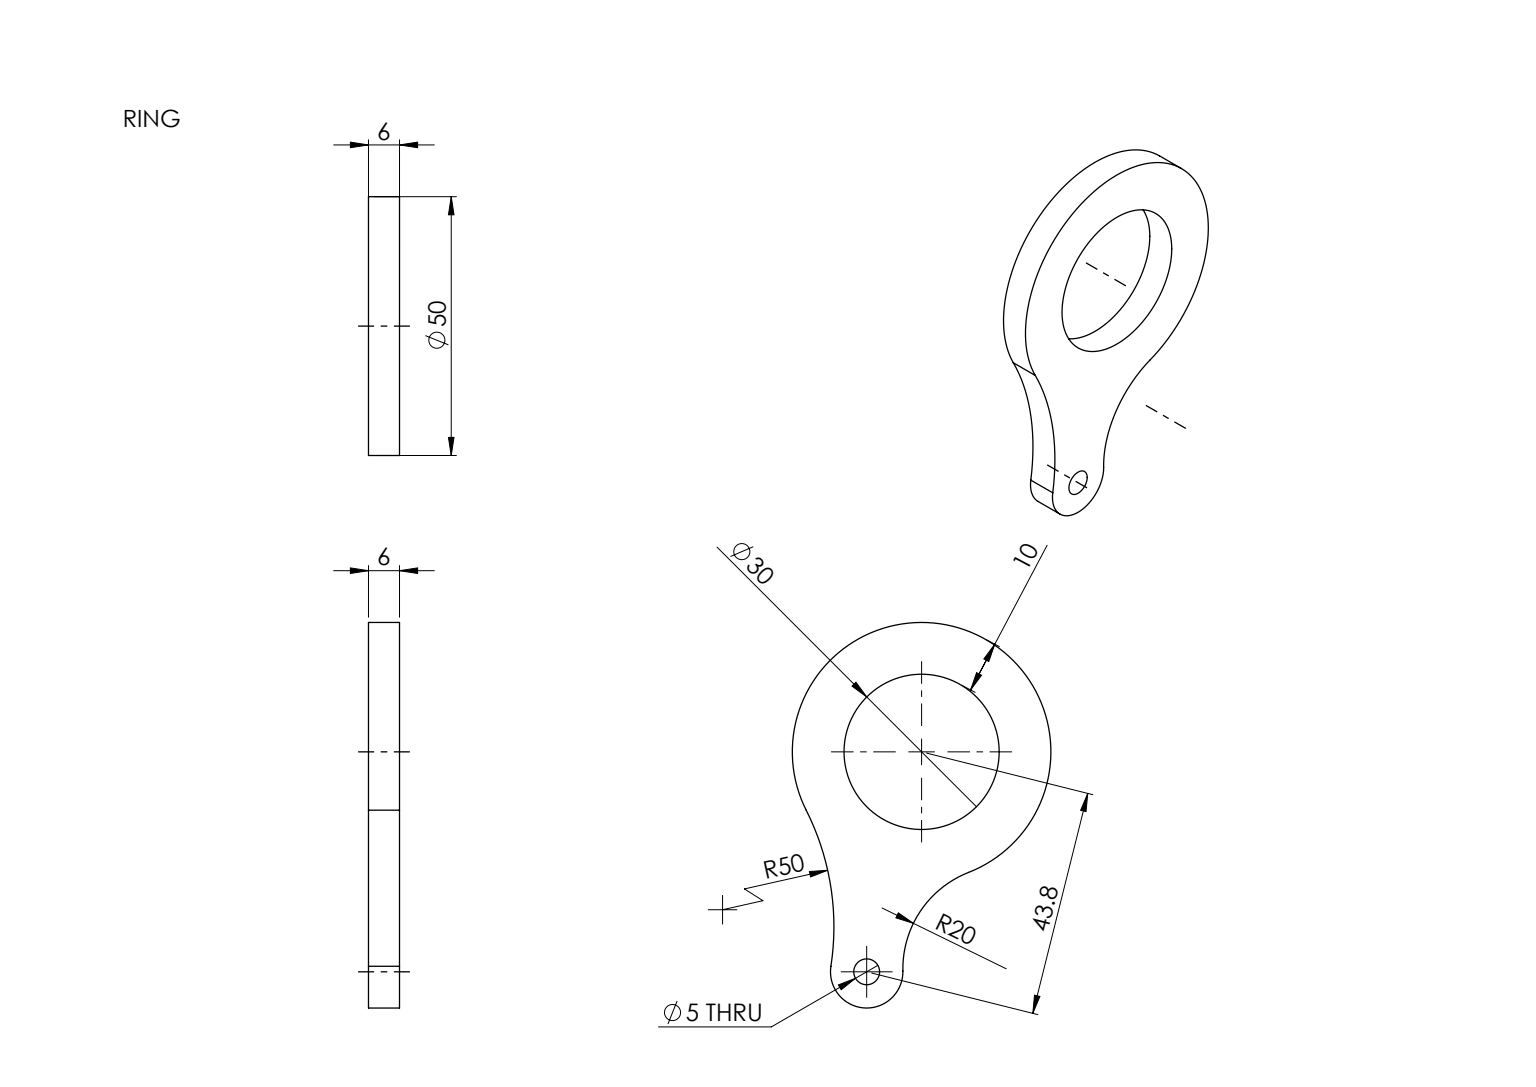
ISO-10303-21;
HEADER;
FILE_DESCRIPTION (('STEP AP214'),
    '1' );
FILE_NAME ('ring.step',
    '2026-10-03T20:08:58',
    ( '' ),
    ( '' ),
    'SwSTEP 2.0',
    'SolidWorks 2026',
    '' );
FILE_SCHEMA (( 'AUTOMOTIVE_DESIGN' ));
ENDSEC;

DATA;
#6=CARTESIAN_POINT ( 'NONE',  ( 33.00000000000001421, 39.34792583643766761, -10.06347054209568270 ) ) ;
#20=( GEOMETRIC_REPRESENTATION_CONTEXT ( 3 ) GLOBAL_UNCERTAINTY_ASSIGNED_CONTEXT ( ( #3670 ) ) GLOBAL_UNIT_ASSIGNED_CONTEXT ( ( #5671, #4709, #1872 ) ) REPRESENTATION_CONTEXT ( 'NONE', 'WORKASPACE' ) );
#46=EDGE_CURVE ( 'NONE', #9407, #3079, #7991, .T. ) ;
#83=ORIENTED_EDGE ( 'NONE', *, *, #1095, .T. ) ;
#164=EDGE_CURVE ( 'NONE', #2848, #3887, #6852, .T. ) ;
#223=EDGE_LOOP ( 'NONE', ( #680, #8634, #6232, #8801 ) ) ;
#258=AXIS2_PLACEMENT_3D ( 'NONE', #11847, #1979, #9819 ) ;
#260=CARTESIAN_POINT ( 'NONE',  ( 33.00000000000001421, 39.34792583643766761, -17.06347054209568270 ) ) ;
#266=DIRECTION ( 'NONE',  ( -1.000000000000000000, 1.006188713385347367E-17, 3.844790828812615713E-17 ) ) ;
#269=EDGE_CURVE ( 'NONE', #1961, #1191, #3966, .T. ) ;
#278=AXIS2_PLACEMENT_3D ( 'NONE', #6450, #2458, #6380 ) ;
#348=ORIENTED_EDGE ( 'NONE', *, *, #8128, .T. ) ;
#366=DIRECTION ( 'NONE',  ( -1.000000000000000000, 1.006188713385347367E-17, 3.844790828812615713E-17 ) ) ;
#371=CARTESIAN_POINT ( 'NONE',  ( 33.00000000000001421, 81.84122341717352356, -52.68198508464163154 ) ) ;
#423=CARTESIAN_POINT ( 'NONE',  ( 33.00000000000000711, 58.55522666905708462, -36.77936687539386185 ) ) ;
#426=DIRECTION ( 'NONE',  ( 1.000000000000000000, -6.162975822039154730E-33, -4.563833282352349791E-17 ) ) ;
#428=ORIENTED_EDGE ( 'NONE', *, *, #736, .F. ) ;
#451=CARTESIAN_POINT ( 'NONE',  ( 33.00000000000001421, 81.84122341717352356, -27.68198508464163510 ) ) ;
#457=ORIENTED_EDGE ( 'NONE', *, *, #9263, .T. ) ;
#554=DIRECTION ( 'NONE',  ( 1.000000000000000000, -6.162975822039154730E-33, -4.563833282352349791E-17 ) ) ;
#581=CARTESIAN_POINT ( 'NONE',  ( 27.00000000000001421, 39.34792583643766761, -17.06347054209568270 ) ) ;
#597=CIRCLE ( 'NONE', #1831, 24.99999999999998934 ) ;
#631=LINE ( 'NONE', #12621, #6264 ) ;
#666=EDGE_CURVE ( 'NONE', #10338, #2092, #3944, .T. ) ;
#676=PLANE ( 'NONE',  #3004 ) ;
#680=ORIENTED_EDGE ( 'NONE', *, *, #6194, .F. ) ;
#735=CYLINDRICAL_SURFACE ( 'NONE', #7583, 19.99999999999999645 ) ;
#736=EDGE_CURVE ( 'NONE', #1153, #9287, #7907, .T. ) ;
#748=EDGE_LOOP ( 'NONE', ( #2877, #7113, #11794, #1502 ) ) ;
#794=CARTESIAN_POINT ( 'NONE',  ( 33.00000000000001421, 40.41548023366553366, -10.14535464186970870 ) ) ;
#795=FACE_BOUND ( 'NONE', #2630, .T. ) ;
#840=EDGE_CURVE ( 'NONE', #1206, #1961, #10652, .T. ) ;
#886=ORIENTED_EDGE ( 'NONE', *, *, #164, .F. ) ;
#890=FACE_OUTER_BOUND ( 'NONE', #6082, .T. ) ;
#900=ORIENTED_EDGE ( 'NONE', *, *, #1095, .F. ) ;
#947=ORIENTED_EDGE ( 'NONE', *, *, #1314, .T. ) ;
#1023=CARTESIAN_POINT ( 'NONE',  ( 33.00000000000000711, 39.92642927056392210, -24.05727230799563898 ) ) ;
#1028=AXIS2_PLACEMENT_3D ( 'NONE', #11252, #426, #7264 ) ;
#1036=LINE ( 'NONE', #4975, #8822 ) ;
#1043=DIRECTION ( 'NONE',  ( 1.000000000000000000, -6.162975822039154730E-33, -4.563833282352349791E-17 ) ) ;
#1082=CIRCLE ( 'NONE', #2757, 19.99999999999998934 ) ;
#1095=EDGE_CURVE ( 'NONE', #3948, #3079, #5308, .T. ) ;
#1107=FACE_OUTER_BOUND ( 'NONE', #1947, .T. ) ;
#1129=ADVANCED_FACE ( 'NONE', ( #11502 ), #735, .F. ) ;
#1153=VERTEX_POINT ( 'NONE', #9602 ) ;
#1170=DIRECTION ( 'NONE',  ( 0.000000000000000000, 0.000000000000000000, -1.000000000000000000 ) ) ;
#1191=VERTEX_POINT ( 'NONE', #794 ) ;
#1206=VERTEX_POINT ( 'NONE', #2693 ) ;
#1215=EDGE_LOOP ( 'NONE', ( #8140, #5838, #6921, #7199 ) ) ;
#1239=CYLINDRICAL_SURFACE ( 'NONE', #2419, 14.99999999999998757 ) ;
#1257=CARTESIAN_POINT ( 'NONE',  ( 27.00000000000001421, 39.49790820824818383, -24.06186359251418594 ) ) ;
#1314=EDGE_CURVE ( 'NONE', #2160, #10794, #1409, .T. ) ;
#1319=DIRECTION ( 'NONE',  ( 0.000000000000000000, 0.000000000000000000, 1.000000000000000000 ) ) ;
#1336=AXIS2_PLACEMENT_3D ( 'NONE', #3651, #3590, #11505 ) ;
#1362=DIRECTION ( 'NONE',  ( 0.000000000000000000, 0.000000000000000000, -1.000000000000000000 ) ) ;
#1372=ORIENTED_EDGE ( 'NONE', *, *, #11676, .T. ) ;
#1383=CARTESIAN_POINT ( 'NONE',  ( 33.00000000000001421, 48.04086878529346194, 39.26975893117280947 ) ) ;
#1409=CIRCLE ( 'NONE', #3880, 2.499999999999992006 ) ;
#1440=ORIENTED_EDGE ( 'NONE', *, *, #12668, .F. ) ;
#1449=CYLINDRICAL_SURFACE ( 'NONE', #6515, 49.99999999999995026 ) ;
#1487=VECTOR ( 'NONE', #10109, 1000.000000000000000 ) ;
#1502=ORIENTED_EDGE ( 'NONE', *, *, #10839, .F. ) ;
#1510=FILL_AREA_STYLE ('',( #7502 ) ) ;
#1512=DIRECTION ( 'NONE',  ( 0.000000000000000000, 0.000000000000000000, 1.000000000000000000 ) ) ;
#1520=DIRECTION ( 'NONE',  ( 0.000000000000000000, 0.000000000000000000, -1.000000000000000000 ) ) ;
#1532=CIRCLE ( 'NONE', #9136, 14.99999999999998934 ) ;
#1539=VECTOR ( 'NONE', #5857, 1000.000000000000000 ) ;
#1606=DIRECTION ( 'NONE',  ( 1.000000000000000000, -6.162975822039154730E-33, -4.563833282352349791E-17 ) ) ;
#1617=AXIS2_PLACEMENT_3D ( 'NONE', #11073, #11142, #1520 ) ;
#1624=DIRECTION ( 'NONE',  ( 0.000000000000000000, 0.000000000000000000, 1.000000000000000000 ) ) ;
#1634=ORIENTED_EDGE ( 'NONE', *, *, #6345, .F. ) ;
#1653=CIRCLE ( 'NONE', #1617, 6.999999999999999112 ) ;
#1671=MECHANICAL_DESIGN_GEOMETRIC_PRESENTATION_REPRESENTATION('',(#4964),#9261);
#1679=DIRECTION ( 'NONE',  ( 1.000000000000000000, -6.162975822039154730E-33, -4.563833282352349791E-17 ) ) ;
#1707=CARTESIAN_POINT ( 'NONE',  ( 27.00000000000001421, 81.84122341717352356, -27.68198508464163510 ) ) ;
#1728=UNCERTAINTY_MEASURE_WITH_UNIT (LENGTH_MEASURE( 1.000000000000000082E-05 ), #6656, 'distance_accuracy_value', 'NONE');
#1732=APPLICATION_CONTEXT ( 'automotive_design' ) ;
#1739=ADVANCED_BREP_SHAPE_REPRESENTATION ( '', ( #5956, #12422 ), #20 ) ;
#1753=DIRECTION ( 'NONE',  ( 0.000000000000000000, 0.000000000000000000, 1.000000000000000000 ) ) ;
#1754=CIRCLE ( 'NONE', #4433, 24.99999999999998934 ) ;
#1825=( LENGTH_UNIT ( ) NAMED_UNIT ( * ) SI_UNIT ( .MILLI., .METRE. ) );
#1831=AXIS2_PLACEMENT_3D ( 'NONE', #8871, #4958, #6761 ) ;
#1872=( NAMED_UNIT ( * ) SI_UNIT ( $, .STERADIAN. ) SOLID_ANGLE_UNIT ( ) );
#1891=DIRECTION ( 'NONE',  ( -4.563833282352349791E-17, 0.000000000000000000, -1.000000000000000000 ) ) ;
#1921=CARTESIAN_POINT ( 'NONE',  ( 33.00000000000001421, 39.34792583643766761, -17.06347054209568270 ) ) ;
#1947=EDGE_LOOP ( 'NONE', ( #8020, #6144, #3063, #8330 ) ) ;
#1957=CARTESIAN_POINT ( 'NONE',  ( 27.00000000000001421, 81.84122341717352356, -27.68198508464163510 ) ) ;
#1959=ORIENTED_EDGE ( 'NONE', *, *, #8551, .T. ) ;
#1961=VERTEX_POINT ( 'NONE', #4156 ) ;
#1979=DIRECTION ( 'NONE',  ( -1.000000000000000000, 6.162975822039154730E-33, 4.563833282352349791E-17 ) ) ;
#2050=EDGE_LOOP ( 'NONE', ( #8866, #9247, #9932, #4731 ) ) ;
#2056=LINE ( 'NONE', #5982, #6902 ) ;
#2089=DIRECTION ( 'NONE',  ( 0.000000000000000000, 0.000000000000000000, -1.000000000000000000 ) ) ;
#2092=VERTEX_POINT ( 'NONE', #9392 ) ;
#2128=CARTESIAN_POINT ( 'NONE',  ( 33.00000000000001421, 39.34792583643766761, -19.56347054209567204 ) ) ;
#2150=DIRECTION ( 'NONE',  ( -1.000000000000000000, 1.006188713385347367E-17, 3.844790828812615713E-17 ) ) ;
#2160=VERTEX_POINT ( 'NONE', #5421 ) ;
#2198=CARTESIAN_POINT ( 'NONE',  ( 33.00000000000001421, 81.84122341717352356, -27.68198508464163510 ) ) ;
#2210=PRODUCT_DEFINITION_FORMATION_WITH_SPECIFIED_SOURCE ( 'ANY', '', #4538, .NOT_KNOWN. ) ;
#2241=EDGE_CURVE ( 'NONE', #4528, #5879, #11115, .T. ) ;
#2250=ORIENTED_EDGE ( 'NONE', *, *, #666, .F. ) ;
#2346=CARTESIAN_POINT ( 'NONE',  ( 27.00000000000001421, 81.84122341717352356, -27.68198508464163510 ) ) ;
#2360=CARTESIAN_POINT ( 'NONE',  ( 33.00000000000001421, 70.57443853988016258, -5.364737079370081041 ) ) ;
#2380=LINE ( 'NONE', #4172, #2959 ) ;
#2412=DIRECTION ( 'NONE',  ( 0.000000000000000000, 0.000000000000000000, 1.000000000000000000 ) ) ;
#2419=AXIS2_PLACEMENT_3D ( 'NONE', #11230, #2150, #2412 ) ;
#2446=LINE ( 'NONE', #11331, #4270 ) ;
#2458=DIRECTION ( 'NONE',  ( -1.000000000000000000, 6.162975822039154730E-33, 4.563833282352349791E-17 ) ) ;
#2539=ORIENTED_EDGE ( 'NONE', *, *, #10803, .F. ) ;
#2548=DIRECTION ( 'NONE',  ( -1.000000000000000000, 1.006188713385347367E-17, 3.844790828812615713E-17 ) ) ;
#2555=DIRECTION ( 'NONE',  ( 0.000000000000000000, 0.000000000000000000, 1.000000000000000000 ) ) ;
#2558=CARTESIAN_POINT ( 'NONE',  ( 33.00000000000001421, -6.037132280312101458E-17, -1.462922435963892052E-15 ) ) ;
#2609=UNCERTAINTY_MEASURE_WITH_UNIT (LENGTH_MEASURE( 1.000000000000000082E-05 ), #1825, 'distance_accuracy_value', 'NONE');
#2630=EDGE_LOOP ( 'NONE', ( #457, #9132 ) ) ;
#2669=EDGE_CURVE ( 'NONE', #7265, #2754, #597, .T. ) ;
#2678=ADVANCED_FACE ( 'NONE', ( #890 ), #10614, .F. ) ;
#2693=CARTESIAN_POINT ( 'NONE',  ( 33.00000000000001421, 81.84122341717352356, -2.681985084641642203 ) ) ;
#2711=EDGE_LOOP ( 'NONE', ( #11837, #7268, #900, #4477 ) ) ;
#2720=ORIENTED_EDGE ( 'NONE', *, *, #840, .F. ) ;
#2726=SHAPE_REPRESENTATION ( 'ring', ( #12422 ), #20 ) ;
#2734=VERTEX_POINT ( 'NONE', #7273 ) ;
#2736=( NAMED_UNIT ( * ) SI_UNIT ( $, .STERADIAN. ) SOLID_ANGLE_UNIT ( ) );
#2738=AXIS2_PLACEMENT_3D ( 'NONE', #4200, #4008, #1170 ) ;
#2754=VERTEX_POINT ( 'NONE', #371 ) ;
#2757=AXIS2_PLACEMENT_3D ( 'NONE', #11977, #10733, #4955 ) ;
#2761=CARTESIAN_POINT ( 'NONE',  ( 27.00000000000001421, -1.664003471950572653E-31, -1.232234986235134900E-15 ) ) ;
#2788=ORIENTED_EDGE ( 'NONE', *, *, #12668, .T. ) ;
#2795=ORIENTED_EDGE ( 'NONE', *, *, #2241, .F. ) ;
#2806=CARTESIAN_POINT ( 'NONE',  ( 33.00000000000001421, 39.34792583643766761, -17.06347054209568270 ) ) ;
#2848=VERTEX_POINT ( 'NONE', #11392 ) ;
#2867=CARTESIAN_POINT ( 'NONE',  ( 27.00000000000001066, 39.92642927056392210, -44.05727230799563898 ) ) ;
#2877=ORIENTED_EDGE ( 'NONE', *, *, #9073, .F. ) ;
#2929=DIRECTION ( 'NONE',  ( -1.000000000000000000, 1.006188713385347367E-17, 3.844790828812615713E-17 ) ) ;
#2959=VECTOR ( 'NONE', #366, 1000.000000000000000 ) ;
#2981=AXIS2_PLACEMENT_3D ( 'NONE', #2867, #7614, #11554 ) ;
#2984=DIRECTION ( 'NONE',  ( 0.000000000000000000, 0.000000000000000000, -1.000000000000000000 ) ) ;
#3004=AXIS2_PLACEMENT_3D ( 'NONE', #2558, #554, #5699 ) ;
#3027=ORIENTED_EDGE ( 'NONE', *, *, #2241, .T. ) ;
#3040=EDGE_CURVE ( 'NONE', #5879, #8571, #4201, .T. ) ;
#3050=CYLINDRICAL_SURFACE ( 'NONE', #12197, 24.99999999999999289 ) ;
#3061=APPLICATION_CONTEXT ( 'automotive_design' ) ;
#3063=ORIENTED_EDGE ( 'NONE', *, *, #6754, .T. ) ;
#3079=VERTEX_POINT ( 'NONE', #8800 ) ;
#3127=CARTESIAN_POINT ( 'NONE',  ( 33.00000000000000711, 39.92642927056392210, -24.05727230799563898 ) ) ;
#3185=DIRECTION ( 'NONE',  ( 0.000000000000000000, 0.000000000000000000, 1.000000000000000000 ) ) ;
#3211=EDGE_LOOP ( 'NONE', ( #2720, #3521, #1959, #7626 ) ) ;
#3269=ORIENTED_EDGE ( 'NONE', *, *, #10839, .T. ) ;
#3353=ORIENTED_EDGE ( 'NONE', *, *, #12439, .F. ) ;
#3398=ORIENTED_EDGE ( 'NONE', *, *, #10467, .F. ) ;
#3451=AXIS2_PLACEMENT_3D ( 'NONE', #2806, #10632, #1753 ) ;
#3456=DIRECTION ( 'NONE',  ( -1.000000000000000000, 1.006188713385347367E-17, 3.844790828812615713E-17 ) ) ;
#3462=AXIS2_PLACEMENT_3D ( 'NONE', #7581, #11525, #6631 ) ;
#3517=CYLINDRICAL_SURFACE ( 'NONE', #8257, 24.99999999999999289 ) ;
#3521=ORIENTED_EDGE ( 'NONE', *, *, #8172, .T. ) ;
#3583=ADVANCED_FACE ( 'NONE', ( #1107 ), #5235, .F. ) ;
#3590=DIRECTION ( 'NONE',  ( -1.000000000000000000, 1.006188713385347367E-17, 3.844790828812615713E-17 ) ) ;
#3631=DIRECTION ( 'NONE',  ( 0.000000000000000000, 0.000000000000000000, -1.000000000000000000 ) ) ;
#3651=CARTESIAN_POINT ( 'NONE',  ( 33.00000000000001421, 39.34792583643766761, -17.06347054209568270 ) ) ;
#3670=UNCERTAINTY_MEASURE_WITH_UNIT (LENGTH_MEASURE( 1.000000000000000082E-05 ), #5671, 'distance_accuracy_value', 'NONE');
#3756=DIRECTION ( 'NONE',  ( 1.000000000000000000, -6.162975822039154730E-33, -4.563833282352349791E-17 ) ) ;
#3769=DIRECTION ( 'NONE',  ( 1.000000000000000000, -6.162975822039154730E-33, -4.563833282352349791E-17 ) ) ;
#3780=VERTEX_POINT ( 'NONE', #9278 ) ;
#3781=ORIENTED_EDGE ( 'NONE', *, *, #8551, .F. ) ;
#3834=AXIS2_PLACEMENT_3D ( 'NONE', #7565, #10323, #1512 ) ;
#3851=DIRECTION ( 'NONE',  ( 0.000000000000000000, 0.000000000000000000, -1.000000000000000000 ) ) ;
#3880=AXIS2_PLACEMENT_3D ( 'NONE', #9858, #1043, #8964 ) ;
#3887=VERTEX_POINT ( 'NONE', #12646 ) ;
#3889=( NAMED_UNIT ( * ) SI_UNIT ( $, .STERADIAN. ) SOLID_ANGLE_UNIT ( ) );
#3917=CIRCLE ( 'NONE', #4535, 24.99999999999998934 ) ;
#3944=CIRCLE ( 'NONE', #7444, 14.99999999999998934 ) ;
#3948=VERTEX_POINT ( 'NONE', #4655 ) ;
#3966=CIRCLE ( 'NONE', #11164, 49.99999999999994316 ) ;
#3969=EDGE_CURVE ( 'NONE', #3079, #4528, #6047, .T. ) ;
#4008=DIRECTION ( 'NONE',  ( -1.000000000000000000, 6.162975822039154730E-33, 4.563833282352349791E-17 ) ) ;
#4047=VECTOR ( 'NONE', #6397, 1000.000000000000000 ) ;
#4156=CARTESIAN_POINT ( 'NONE',  ( 33.00000000000001421, 70.57443853988016258, -5.364737079370081041 ) ) ;
#4172=CARTESIAN_POINT ( 'NONE',  ( 33.00000000000001421, 39.34792583643766761, -19.56347054209567204 ) ) ;
#4200=CARTESIAN_POINT ( 'NONE',  ( 33.00000000000001421, 39.34792583643766761, -17.06347054209568270 ) ) ;
#4201=CIRCLE ( 'NONE', #12027, 6.999999999999999112 ) ;
#4261=AXIS2_PLACEMENT_3D ( 'NONE', #260, #7098, #3185 ) ;
#4263=DIRECTION ( 'NONE',  ( -1.000000000000000000, 1.006188713385347367E-17, 3.844790828812615713E-17 ) ) ;
#4266=ADVANCED_FACE ( 'NONE', ( #4627 ), #8547, .F. ) ;
#4270=VECTOR ( 'NONE', #6881, 1000.000000000000000 ) ;
#4275=LINE ( 'NONE', #2360, #9888 ) ;
#4283=EDGE_CURVE ( 'NONE', #9287, #5879, #2446, .T. ) ;
#4315=VECTOR ( 'NONE', #266, 1000.000000000000000 ) ;
#4341=ORIENTED_EDGE ( 'NONE', *, *, #164, .T. ) ;
#4381=CIRCLE ( 'NONE', #258, 6.999999999999999112 ) ;
#4405=ORIENTED_EDGE ( 'NONE', *, *, #840, .T. ) ;
#4433=AXIS2_PLACEMENT_3D ( 'NONE', #1707, #6549, #7636 ) ;
#4458=MECHANICAL_DESIGN_GEOMETRIC_PRESENTATION_REPRESENTATION('',(#7344),#10617);
#4477=ORIENTED_EDGE ( 'NONE', *, *, #4523, .F. ) ;
#4481=PRESENTATION_STYLE_ASSIGNMENT (( #9352 ) ) ;
#4493=VERTEX_POINT ( 'NONE', #8150 ) ;
#4523=EDGE_CURVE ( 'NONE', #7265, #3948, #11899, .T. ) ;
#4528=VERTEX_POINT ( 'NONE', #1257 ) ;
#4535=AXIS2_PLACEMENT_3D ( 'NONE', #9705, #7026, #2984 ) ;
#4538=PRODUCT ( 'ring', 'ring', '', ( #10781 ) ) ;
#4548=SURFACE_STYLE_FILL_AREA ( #1510 ) ;
#4619=EDGE_LOOP ( 'NONE', ( #4341, #12276 ) ) ;
#4627=FACE_OUTER_BOUND ( 'NONE', #2711, .T. ) ;
#4655=CARTESIAN_POINT ( 'NONE',  ( 27.00000000000001066, 58.55522666905708462, -36.77936687539386185 ) ) ;
#4660=ADVANCED_FACE ( 'NONE', ( #7445 ), #6613, .F. ) ;
#4671=AXIS2_PLACEMENT_3D ( 'NONE', #8322, #10306, #1624 ) ;
#4672=FACE_BOUND ( 'NONE', #4619, .T. ) ;
#4709=( NAMED_UNIT ( * ) PLANE_ANGLE_UNIT ( ) SI_UNIT ( $, .RADIAN. ) );
#4729=AXIS2_PLACEMENT_3D ( 'NONE', #11567, #3769, #8401 ) ;
#4731=ORIENTED_EDGE ( 'NONE', *, *, #8172, .F. ) ;
#4777=DIRECTION ( 'NONE',  ( 0.000000000000000000, 6.839766848137126197E-14, -1.000000000000000000 ) ) ;
#4824=ADVANCED_FACE ( 'NONE', ( #4672, #8724, #795 ), #7876, .F. ) ;
#4955=DIRECTION ( 'NONE',  ( 0.000000000000000000, 0.000000000000000000, -1.000000000000000000 ) ) ;
#4958=DIRECTION ( 'NONE',  ( 1.000000000000000000, -6.162975822039154730E-33, -4.563833282352349791E-17 ) ) ;
#4964=STYLED_ITEM ( 'NONE', ( #10686 ), #1739 ) ;
#4975=CARTESIAN_POINT ( 'NONE',  ( 33.00000000000001421, 39.34792583643766761, -10.06347054209568270 ) ) ;
#4991=EDGE_LOOP ( 'NONE', ( #83, #12550, #3027, #8078, #3269, #1634, #3781, #2539, #9178 ) ) ;
#5037=DIRECTION ( 'NONE',  ( 0.000000000000000000, 0.000000000000000000, -1.000000000000000000 ) ) ;
#5039=AXIS2_PLACEMENT_3D ( 'NONE', #8359, #9313, #8423 ) ;
#5048=CARTESIAN_POINT ( 'NONE',  ( 33.00000000000001421, 81.84122341717352356, -27.68198508464163510 ) ) ;
#5049=FACE_OUTER_BOUND ( 'NONE', #7186, .T. ) ;
#5055=CARTESIAN_POINT ( 'NONE',  ( 27.00000000000001421, 39.34792583643766761, -10.06347054209568270 ) ) ;
#5098=ADVANCED_FACE ( 'NONE', ( #11426 ), #10442, .T. ) ;
#5164=PRODUCT_DEFINITION ( 'UNKNOWN', '', #2210, #9661 ) ;
#5179=CARTESIAN_POINT ( 'NONE',  ( 33.00000000000001421, 40.41548023366553366, -10.14535464186970870 ) ) ;
#5203=AXIS2_PLACEMENT_3D ( 'NONE', #8158, #5205, #10269 ) ;
#5205=DIRECTION ( 'NONE',  ( 1.000000000000000000, -6.162975822039154730E-33, -4.563833282352349791E-17 ) ) ;
#5209=EDGE_LOOP ( 'NONE', ( #2250, #11125 ) ) ;
#5235=CYLINDRICAL_SURFACE ( 'NONE', #6242, 14.99999999999998757 ) ;
#5260=ADVANCED_FACE ( 'NONE', ( #12648 ), #8580, .T. ) ;
#5308=CIRCLE ( 'NONE', #4729, 19.99999999999998934 ) ;
#5403=VERTEX_POINT ( 'NONE', #9843 ) ;
#5420=ADVANCED_FACE ( 'NONE', ( #11993 ), #8887, .T. ) ;
#5421=CARTESIAN_POINT ( 'NONE',  ( 33.00000000000001421, 39.34792583643766761, -14.56347054209569158 ) ) ;
#5534=ORIENTED_EDGE ( 'NONE', *, *, #3040, .F. ) ;
#5546=CARTESIAN_POINT ( 'NONE',  ( 33.00000000000001421, 39.34792583643766761, -24.06347054209567915 ) ) ;
#5633=FACE_OUTER_BOUND ( 'NONE', #6455, .T. ) ;
#5671=( LENGTH_UNIT ( ) NAMED_UNIT ( * ) SI_UNIT ( .MILLI., .METRE. ) );
#5699=DIRECTION ( 'NONE',  ( -4.563833282352349791E-17, 0.000000000000000000, -1.000000000000000000 ) ) ;
#5707=CARTESIAN_POINT ( 'NONE',  ( 0.000000000000000000, 0.000000000000000000, 0.000000000000000000 ) ) ;
#5725=ADVANCED_FACE ( 'NONE', ( #6340 ), #1449, .F. ) ;
#5838=ORIENTED_EDGE ( 'NONE', *, *, #9824, .T. ) ;
#5857=DIRECTION ( 'NONE',  ( -1.000000000000000000, 1.006188713385347367E-17, 3.844790828812615713E-17 ) ) ;
#5879=VERTEX_POINT ( 'NONE', #10388 ) ;
#5891=COLOUR_RGB ( '', 0.08235294, 0.09019608, 0.10196078) ;
#5903=ORIENTED_EDGE ( 'NONE', *, *, #12657, .F. ) ;
#5925=DIRECTION ( 'NONE',  ( -1.000000000000000000, 6.162975822039154730E-33, 4.563833282352349791E-17 ) ) ;
#5941=DIRECTION ( 'NONE',  ( 0.000000000000000000, 0.000000000000000000, 1.000000000000000000 ) ) ;
#5956=MANIFOLD_SOLID_BREP ( 'Boss-Extrude1', #9901 ) ;
#5982=CARTESIAN_POINT ( 'NONE',  ( 33.00000000000001421, 81.84122341717352356, -2.681985084641642203 ) ) ;
#5994=DIRECTION ( 'NONE',  ( 1.000000000000000000, -6.162975822039154730E-33, -4.563833282352349791E-17 ) ) ;
#6047=CIRCLE ( 'NONE', #2981, 19.99999999999998934 ) ;
#6082=EDGE_LOOP ( 'NONE', ( #947, #2788, #6163, #8928 ) ) ;
#6123=ADVANCED_FACE ( 'NONE', ( #5049 ), #1239, .F. ) ;
#6144=ORIENTED_EDGE ( 'NONE', *, *, #7752, .T. ) ;
#6163=ORIENTED_EDGE ( 'NONE', *, *, #9263, .F. ) ;
#6194=EDGE_CURVE ( 'NONE', #2754, #10809, #7549, .T. ) ;
#6224=AXIS2_PLACEMENT_3D ( 'NONE', #2346, #10170, #1362 ) ;
#6232=ORIENTED_EDGE ( 'NONE', *, *, #4523, .T. ) ;
#6242=AXIS2_PLACEMENT_3D ( 'NONE', #5048, #10895, #5941 ) ;
#6264=VECTOR ( 'NONE', #10604, 1000.000000000000000 ) ;
#6317=EDGE_CURVE ( 'NONE', #10794, #2160, #8575, .T. ) ;
#6340=FACE_OUTER_BOUND ( 'NONE', #11330, .T. ) ;
#6345=EDGE_CURVE ( 'NONE', #4493, #2734, #10626, .T. ) ;
#6380=DIRECTION ( 'NONE',  ( 0.000000000000000000, 6.839766848137126197E-14, -1.000000000000000000 ) ) ;
#6386=AXIS2_PLACEMENT_3D ( 'NONE', #10347, #9375, #9315 ) ;
#6397=DIRECTION ( 'NONE',  ( -1.000000000000000000, 1.006188713385347367E-17, 3.844790828812615713E-17 ) ) ;
#6428=DIRECTION ( 'NONE',  ( 1.000000000000000000, 0.000000000000000000, 0.000000000000000000 ) ) ;
#6449=EDGE_CURVE ( 'NONE', #3887, #2848, #8107, .T. ) ;
#6450=CARTESIAN_POINT ( 'NONE',  ( 33.00000000000001421, 39.34792583643766761, -17.06347054209568270 ) ) ;
#6455=EDGE_LOOP ( 'NONE', ( #3353, #12393, #11072, #4405, #7881, #9758, #10702, #428, #12101 ) ) ;
#6515=AXIS2_PLACEMENT_3D ( 'NONE', #1383, #9048, #1319 ) ;
#6528=DIRECTION ( 'NONE',  ( -1.000000000000000000, 6.162975822039154730E-33, 4.563833282352349791E-17 ) ) ;
#6549=DIRECTION ( 'NONE',  ( 1.000000000000000000, -6.162975822039154730E-33, -4.563833282352349791E-17 ) ) ;
#6613=CYLINDRICAL_SURFACE ( 'NONE', #3834, 2.499999999999990230 ) ;
#6614=ORIENTED_EDGE ( 'NONE', *, *, #9073, .T. ) ;
#6631=DIRECTION ( 'NONE',  ( 0.000000000000000000, 0.000000000000000000, 1.000000000000000000 ) ) ;
#6656=( LENGTH_UNIT ( ) NAMED_UNIT ( * ) SI_UNIT ( .MILLI., .METRE. ) );
#6692=CARTESIAN_POINT ( 'NONE',  ( 27.00000000000001421, 39.34792583643766761, -17.06347054209568270 ) ) ;
#6737=FACE_BOUND ( 'NONE', #5209, .T. ) ;
#6754=EDGE_CURVE ( 'NONE', #10338, #2848, #631, .T. ) ;
#6761=DIRECTION ( 'NONE',  ( 0.000000000000000000, 0.000000000000000000, -1.000000000000000000 ) ) ;
#6764=DIRECTION ( 'NONE',  ( 1.000000000000000000, -6.162975822039154730E-33, -4.563833282352349791E-17 ) ) ;
#6774=SURFACE_STYLE_USAGE ( .BOTH. , #12706 ) ;
#6852=CIRCLE ( 'NONE', #6224, 14.99999999999998934 ) ;
#6881=DIRECTION ( 'NONE',  ( -1.000000000000000000, 1.006188713385347367E-17, 3.844790828812615713E-17 ) ) ;
#6902=VECTOR ( 'NONE', #8939, 1000.000000000000000 ) ;
#6912=CARTESIAN_POINT ( 'NONE',  ( 33.00000000000001421, 81.84122341717352356, -27.68198508464163510 ) ) ;
#6921=ORIENTED_EDGE ( 'NONE', *, *, #10467, .T. ) ;
#6928=AXIS2_PLACEMENT_3D ( 'NONE', #2761, #8592, #1891 ) ;
#7026=DIRECTION ( 'NONE',  ( 1.000000000000000000, -6.162975822039154730E-33, -4.563833282352349791E-17 ) ) ;
#7037=CARTESIAN_POINT ( 'NONE',  ( 33.00000000000001421, 81.84122341717352356, -12.68198508464164931 ) ) ;
#7051=DIRECTION ( 'NONE',  ( 1.000000000000000000, -6.162975822039154730E-33, -4.563833282352349791E-17 ) ) ;
#7053=ADVANCED_FACE ( 'NONE', ( #6737, #5633, #10524 ), #676, .T. ) ;
#7098=DIRECTION ( 'NONE',  ( -1.000000000000000000, 1.006188713385347367E-17, 3.844790828812615713E-17 ) ) ;
#7109=ADVANCED_FACE ( 'NONE', ( #12606 ), #12414, .T. ) ;
#7113=ORIENTED_EDGE ( 'NONE', *, *, #12484, .T. ) ;
#7122=SHAPE_DEFINITION_REPRESENTATION ( #8228, #2726 ) ;
#7128=EDGE_CURVE ( 'NONE', #3948, #10809, #1754, .T. ) ;
#7151=AXIS2_PLACEMENT_3D ( 'NONE', #10753, #3756, #9590 ) ;
#7186=EDGE_LOOP ( 'NONE', ( #7630, #348, #886, #12201 ) ) ;
#7199=ORIENTED_EDGE ( 'NONE', *, *, #3969, .F. ) ;
#7216=CIRCLE ( 'NONE', #1028, 19.99999999999998934 ) ;
#7264=DIRECTION ( 'NONE',  ( 0.000000000000000000, 0.000000000000000000, -1.000000000000000000 ) ) ;
#7265=VERTEX_POINT ( 'NONE', #9863 ) ;
#7268=ORIENTED_EDGE ( 'NONE', *, *, #46, .T. ) ;
#7273=CARTESIAN_POINT ( 'NONE',  ( 27.00000000000001421, 40.41548023366553366, -10.14535464186970870 ) ) ;
#7344=STYLED_ITEM ( 'NONE', ( #4481 ), #5956 ) ;
#7345=EDGE_LOOP ( 'NONE', ( #9744, #9259, #2795, #3398 ) ) ;
#7391=EDGE_CURVE ( 'NONE', #1191, #2734, #10175, .T. ) ;
#7392=DIRECTION ( 'NONE',  ( 0.000000000000000000, 0.000000000000000000, 1.000000000000000000 ) ) ;
#7423=LINE ( 'NONE', #10298, #11573 ) ;
#7444=AXIS2_PLACEMENT_3D ( 'NONE', #451, #1606, #9513 ) ;
#7445=FACE_OUTER_BOUND ( 'NONE', #9112, .T. ) ;
#7502=FILL_AREA_STYLE_COLOUR ( '', #5891 ) ;
#7549=LINE ( 'NONE', #11555, #4047 ) ;
#7565=CARTESIAN_POINT ( 'NONE',  ( 33.00000000000001421, 39.34792583643766761, -17.06347054209568270 ) ) ;
#7581=CARTESIAN_POINT ( 'NONE',  ( 33.00000000000000711, 39.92642927056392210, -44.05727230799563898 ) ) ;
#7583=AXIS2_PLACEMENT_3D ( 'NONE', #11376, #8462, #2555 ) ;
#7597=CARTESIAN_POINT ( 'NONE',  ( 33.00000000000001421, 81.84122341717352356, -27.68198508464163510 ) ) ;
#7614=DIRECTION ( 'NONE',  ( 1.000000000000000000, -6.162975822039154730E-33, -4.563833282352349791E-17 ) ) ;
#7626=ORIENTED_EDGE ( 'NONE', *, *, #11251, .F. ) ;
#7630=ORIENTED_EDGE ( 'NONE', *, *, #666, .T. ) ;
#7636=DIRECTION ( 'NONE',  ( 0.000000000000000000, 0.000000000000000000, -1.000000000000000000 ) ) ;
#7697=CIRCLE ( 'NONE', #11201, 24.99999999999998934 ) ;
#7747=DIRECTION ( 'NONE',  ( -1.000000000000000000, 1.006188713385347367E-17, 3.844790828812615713E-17 ) ) ;
#7752=EDGE_CURVE ( 'NONE', #2092, #10338, #1532, .T. ) ;
#7786=DIRECTION ( 'NONE',  ( 0.000000000000000000, 0.000000000000000000, 1.000000000000000000 ) ) ;
#7788=DIRECTION ( 'NONE',  ( 0.000000000000000000, 0.000000000000000000, -1.000000000000000000 ) ) ;
#7793=CARTESIAN_POINT ( 'NONE',  ( 27.00000000000001421, 81.84122341717352356, -52.68198508464163154 ) ) ;
#7876=PLANE ( 'NONE',  #6928 ) ;
#7881=ORIENTED_EDGE ( 'NONE', *, *, #269, .T. ) ;
#7889=DIRECTION ( 'NONE',  ( -1.000000000000000000, 6.162975822039154730E-33, 4.563833282352349791E-17 ) ) ;
#7907=CIRCLE ( 'NONE', #278, 6.999999999999999112 ) ;
#7991=LINE ( 'NONE', #3127, #1487 ) ;
#8020=ORIENTED_EDGE ( 'NONE', *, *, #8128, .F. ) ;
#8078=ORIENTED_EDGE ( 'NONE', *, *, #3040, .T. ) ;
#8107=CIRCLE ( 'NONE', #5039, 14.99999999999998934 ) ;
#8128=EDGE_CURVE ( 'NONE', #2092, #3887, #10618, .T. ) ;
#8140=ORIENTED_EDGE ( 'NONE', *, *, #46, .F. ) ;
#8150=CARTESIAN_POINT ( 'NONE',  ( 27.00000000000001421, 70.57443853988016258, -5.364737079370081041 ) ) ;
#8158=CARTESIAN_POINT ( 'NONE',  ( 27.00000000000001421, 39.34792583643766761, -17.06347054209568270 ) ) ;
#8172=EDGE_CURVE ( 'NONE', #1206, #5403, #2056, .T. ) ;
#8228=PRODUCT_DEFINITION_SHAPE ( 'NONE', 'NONE',  #5164 ) ;
#8257=AXIS2_PLACEMENT_3D ( 'NONE', #11366, #2548, #10379 ) ;
#8314=LINE ( 'NONE', #9147, #4315 ) ;
#8322=CARTESIAN_POINT ( 'NONE',  ( 33.00000000000001421, 81.84122341717352356, -27.68198508464163510 ) ) ;
#8330=ORIENTED_EDGE ( 'NONE', *, *, #6449, .F. ) ;
#8359=CARTESIAN_POINT ( 'NONE',  ( 27.00000000000001421, 81.84122341717352356, -27.68198508464163510 ) ) ;
#8364=ORIENTED_EDGE ( 'NONE', *, *, #269, .F. ) ;
#8401=DIRECTION ( 'NONE',  ( 0.000000000000000000, 0.000000000000000000, -1.000000000000000000 ) ) ;
#8423=DIRECTION ( 'NONE',  ( 0.000000000000000000, 0.000000000000000000, -1.000000000000000000 ) ) ;
#8433=CIRCLE ( 'NONE', #6386, 24.99999999999998934 ) ;
#8461=SURFACE_SIDE_STYLE ('',( #4548 ) ) ;
#8462=DIRECTION ( 'NONE',  ( -1.000000000000000000, 1.006188713385347367E-17, 3.844790828812615713E-17 ) ) ;
#8508=CARTESIAN_POINT ( 'NONE',  ( 33.00000000000001421, 48.04086878529346194, 39.26975893117280947 ) ) ;
#8547=CYLINDRICAL_SURFACE ( 'NONE', #3462, 19.99999999999999645 ) ;
#8551=EDGE_CURVE ( 'NONE', #5403, #4493, #7697, .T. ) ;
#8571=VERTEX_POINT ( 'NONE', #5055 ) ;
#8575=CIRCLE ( 'NONE', #7151, 2.499999999999992006 ) ;
#8580=CYLINDRICAL_SURFACE ( 'NONE', #3451, 6.999999999999999112 ) ;
#8592=DIRECTION ( 'NONE',  ( 1.000000000000000000, -6.162975822039154730E-33, -4.563833282352349791E-17 ) ) ;
#8634=ORIENTED_EDGE ( 'NONE', *, *, #2669, .F. ) ;
#8660=( NAMED_UNIT ( * ) PLANE_ANGLE_UNIT ( ) SI_UNIT ( $, .RADIAN. ) );
#8705=FILL_AREA_STYLE ('',( #8763 ) ) ;
#8724=FACE_OUTER_BOUND ( 'NONE', #4991, .T. ) ;
#8752=DIRECTION ( 'NONE',  ( -1.000000000000000000, 1.006188713385347367E-17, 3.844790828812615713E-17 ) ) ;
#8763=FILL_AREA_STYLE_COLOUR ( '', #12379 ) ;
#8800=CARTESIAN_POINT ( 'NONE',  ( 27.00000000000001066, 39.92642927056392210, -24.05727230799563898 ) ) ;
#8801=ORIENTED_EDGE ( 'NONE', *, *, #7128, .T. ) ;
#8822=VECTOR ( 'NONE', #7747, 1000.000000000000000 ) ;
#8825=DIRECTION ( 'NONE',  ( -6.938893903907235773E-17, 0.000000000000000000, -1.000000000000000000 ) ) ;
#8866=ORIENTED_EDGE ( 'NONE', *, *, #9651, .F. ) ;
#8871=CARTESIAN_POINT ( 'NONE',  ( 33.00000000000001421, 81.84122341717352356, -27.68198508464163510 ) ) ;
#8876=CARTESIAN_POINT ( 'NONE',  ( 33.00000000000001421, 81.84122341717352356, -42.68198508464162444 ) ) ;
#8887=CYLINDRICAL_SURFACE ( 'NONE', #4261, 6.999999999999999112 ) ;
#8928=ORIENTED_EDGE ( 'NONE', *, *, #11767, .F. ) ;
#8939=DIRECTION ( 'NONE',  ( -1.000000000000000000, 1.006188713385347367E-17, 3.844790828812615713E-17 ) ) ;
#8964=DIRECTION ( 'NONE',  ( 0.000000000000000000, 0.000000000000000000, -1.000000000000000000 ) ) ;
#9044=AXIS2_PLACEMENT_3D ( 'NONE', #10749, #5925, #4777 ) ;
#9048=DIRECTION ( 'NONE',  ( -1.000000000000000000, 1.006188713385347367E-17, 3.844790828812615713E-17 ) ) ;
#9054=ORIENTED_EDGE ( 'NONE', *, *, #11251, .T. ) ;
#9073=EDGE_CURVE ( 'NONE', #12081, #8571, #1036, .T. ) ;
#9112=EDGE_LOOP ( 'NONE', ( #1440, #11130, #10050, #5903 ) ) ;
#9132=ORIENTED_EDGE ( 'NONE', *, *, #12657, .T. ) ;
#9136=AXIS2_PLACEMENT_3D ( 'NONE', #6912, #5994, #5037 ) ;
#9147=CARTESIAN_POINT ( 'NONE',  ( 33.00000000000001421, 39.49790820824818383, -24.06186359251418594 ) ) ;
#9178=ORIENTED_EDGE ( 'NONE', *, *, #7128, .F. ) ;
#9247=ORIENTED_EDGE ( 'NONE', *, *, #6194, .T. ) ;
#9259=ORIENTED_EDGE ( 'NONE', *, *, #4283, .T. ) ;
#9261=( GEOMETRIC_REPRESENTATION_CONTEXT ( 3 ) GLOBAL_UNCERTAINTY_ASSIGNED_CONTEXT ( ( #1728 ) ) GLOBAL_UNIT_ASSIGNED_CONTEXT ( ( #6656, #9711, #2736 ) ) REPRESENTATION_CONTEXT ( 'NONE', 'WORKASPACE' ) );
#9263=EDGE_CURVE ( 'NONE', #10485, #3780, #11089, .T. ) ;
#9278=CARTESIAN_POINT ( 'NONE',  ( 27.00000000000001421, 39.34792583643766761, -19.56347054209567204 ) ) ;
#9287=VERTEX_POINT ( 'NONE', #5546 ) ;
#9313=DIRECTION ( 'NONE',  ( 1.000000000000000000, -6.162975822039154730E-33, -4.563833282352349791E-17 ) ) ;
#9315=DIRECTION ( 'NONE',  ( 0.000000000000000000, 0.000000000000000000, -1.000000000000000000 ) ) ;
#9352=SURFACE_STYLE_USAGE ( .BOTH. , #8461 ) ;
#9375=DIRECTION ( 'NONE',  ( 1.000000000000000000, -6.162975822039154730E-33, -4.563833282352349791E-17 ) ) ;
#9392=CARTESIAN_POINT ( 'NONE',  ( 33.00000000000001421, 81.84122341717352356, -42.68198508464162444 ) ) ;
#9407=VERTEX_POINT ( 'NONE', #1023 ) ;
#9513=DIRECTION ( 'NONE',  ( 0.000000000000000000, 0.000000000000000000, -1.000000000000000000 ) ) ;
#9590=DIRECTION ( 'NONE',  ( 0.000000000000000000, 0.000000000000000000, -1.000000000000000000 ) ) ;
#9602=CARTESIAN_POINT ( 'NONE',  ( 33.00000000000001421, 39.49790820824818383, -24.06186359251418594 ) ) ;
#9651=EDGE_CURVE ( 'NONE', #2754, #1206, #8433, .T. ) ;
#9661=PRODUCT_DEFINITION_CONTEXT ( 'detailed design', #3061, 'design' ) ;
#9705=CARTESIAN_POINT ( 'NONE',  ( 27.00000000000001421, 81.84122341717352356, -27.68198508464163510 ) ) ;
#9711=( NAMED_UNIT ( * ) PLANE_ANGLE_UNIT ( ) SI_UNIT ( $, .RADIAN. ) );
#9744=ORIENTED_EDGE ( 'NONE', *, *, #736, .T. ) ;
#9758=ORIENTED_EDGE ( 'NONE', *, *, #12484, .F. ) ;
#9819=DIRECTION ( 'NONE',  ( 0.000000000000000000, 0.000000000000000000, -1.000000000000000000 ) ) ;
#9824=EDGE_CURVE ( 'NONE', #9407, #1153, #7216, .T. ) ;
#9835=DIRECTION ( 'NONE',  ( 0.000000000000000000, 0.000000000000000000, 1.000000000000000000 ) ) ;
#9843=CARTESIAN_POINT ( 'NONE',  ( 27.00000000000001421, 81.84122341717352356, -2.681985084641642203 ) ) ;
#9858=CARTESIAN_POINT ( 'NONE',  ( 33.00000000000001421, 39.34792583643766761, -17.06347054209568270 ) ) ;
#9863=CARTESIAN_POINT ( 'NONE',  ( 33.00000000000000711, 58.55522666905708462, -36.77936687539386185 ) ) ;
#9883=ORIENTED_EDGE ( 'NONE', *, *, #4283, .F. ) ;
#9888=VECTOR ( 'NONE', #3456, 1000.000000000000000 ) ;
#9901=CLOSED_SHELL ( 'NONE', ( #2678, #6123, #7109, #5420, #12038, #5098, #4266, #1129, #11354, #5725, #5260, #3583, #4660, #7053, #4824 ) ) ;
#9932=ORIENTED_EDGE ( 'NONE', *, *, #10803, .T. ) ;
#9993=ORIENTED_EDGE ( 'NONE', *, *, #7391, .F. ) ;
#10043=AXIS2_PLACEMENT_3D ( 'NONE', #1921, #8752, #7786 ) ;
#10050=ORIENTED_EDGE ( 'NONE', *, *, #11767, .T. ) ;
#10109=DIRECTION ( 'NONE',  ( -1.000000000000000000, 1.006188713385347367E-17, 3.844790828812615713E-17 ) ) ;
#10170=DIRECTION ( 'NONE',  ( 1.000000000000000000, -6.162975822039154730E-33, -4.563833282352349791E-17 ) ) ;
#10175=LINE ( 'NONE', #5179, #11227 ) ;
#10197=ORIENTED_EDGE ( 'NONE', *, *, #6345, .T. ) ;
#10269=DIRECTION ( 'NONE',  ( 0.000000000000000000, 0.000000000000000000, -1.000000000000000000 ) ) ;
#10298=CARTESIAN_POINT ( 'NONE',  ( 33.00000000000001421, 39.34792583643766761, -14.56347054209569158 ) ) ;
#10306=DIRECTION ( 'NONE',  ( -1.000000000000000000, 1.006188713385347367E-17, 3.844790828812615713E-17 ) ) ;
#10323=DIRECTION ( 'NONE',  ( -1.000000000000000000, 1.006188713385347367E-17, 3.844790828812615713E-17 ) ) ;
#10338=VERTEX_POINT ( 'NONE', #7037 ) ;
#10347=CARTESIAN_POINT ( 'NONE',  ( 33.00000000000001421, 81.84122341717352356, -27.68198508464163510 ) ) ;
#10379=DIRECTION ( 'NONE',  ( 0.000000000000000000, 0.000000000000000000, 1.000000000000000000 ) ) ;
#10388=CARTESIAN_POINT ( 'NONE',  ( 27.00000000000001421, 39.34792583643766761, -24.06347054209567915 ) ) ;
#10442=CYLINDRICAL_SURFACE ( 'NONE', #4671, 24.99999999999999289 ) ;
#10467=EDGE_CURVE ( 'NONE', #1153, #4528, #8314, .T. ) ;
#10485=VERTEX_POINT ( 'NONE', #12194 ) ;
#10524=FACE_BOUND ( 'NONE', #12542, .T. ) ;
#10604=DIRECTION ( 'NONE',  ( -1.000000000000000000, 1.006188713385347367E-17, 3.844790828812615713E-17 ) ) ;
#10614=CYLINDRICAL_SURFACE ( 'NONE', #10043, 2.499999999999990230 ) ;
#10617=( GEOMETRIC_REPRESENTATION_CONTEXT ( 3 ) GLOBAL_UNCERTAINTY_ASSIGNED_CONTEXT ( ( #2609 ) ) GLOBAL_UNIT_ASSIGNED_CONTEXT ( ( #1825, #8660, #3889 ) ) REPRESENTATION_CONTEXT ( 'NONE', 'WORKASPACE' ) );
#10618=LINE ( 'NONE', #8876, #1539 ) ;
#10626=CIRCLE ( 'NONE', #11260, 49.99999999999994316 ) ;
#10632=DIRECTION ( 'NONE',  ( -1.000000000000000000, 1.006188713385347367E-17, 3.844790828812615713E-17 ) ) ;
#10652=CIRCLE ( 'NONE', #10856, 24.99999999999998934 ) ;
#10686=PRESENTATION_STYLE_ASSIGNMENT (( #6774 ) ) ;
#10702=ORIENTED_EDGE ( 'NONE', *, *, #11676, .F. ) ;
#10733=DIRECTION ( 'NONE',  ( 1.000000000000000000, -6.162975822039154730E-33, -4.563833282352349791E-17 ) ) ;
#10739=CIRCLE ( 'NONE', #5203, 2.499999999999992006 ) ;
#10749=CARTESIAN_POINT ( 'NONE',  ( 27.00000000000001421, 39.34792583643766761, -17.06347054209568270 ) ) ;
#10753=CARTESIAN_POINT ( 'NONE',  ( 33.00000000000001421, 39.34792583643766761, -17.06347054209568270 ) ) ;
#10781=PRODUCT_CONTEXT ( 'NONE', #1732, 'mechanical' ) ;
#10794=VERTEX_POINT ( 'NONE', #2128 ) ;
#10803=EDGE_CURVE ( 'NONE', #10809, #5403, #3917, .T. ) ;
#10809=VERTEX_POINT ( 'NONE', #7793 ) ;
#10837=VECTOR ( 'NONE', #12162, 1000.000000000000000 ) ;
#10839=EDGE_CURVE ( 'NONE', #8571, #2734, #1653, .T. ) ;
#10856=AXIS2_PLACEMENT_3D ( 'NONE', #7597, #6764, #7788 ) ;
#10895=DIRECTION ( 'NONE',  ( -1.000000000000000000, 1.006188713385347367E-17, 3.844790828812615713E-17 ) ) ;
#11009=ORIENTED_EDGE ( 'NONE', *, *, #1314, .F. ) ;
#11072=ORIENTED_EDGE ( 'NONE', *, *, #9651, .T. ) ;
#11073=CARTESIAN_POINT ( 'NONE',  ( 27.00000000000001421, 39.34792583643766761, -17.06347054209568270 ) ) ;
#11089=CIRCLE ( 'NONE', #11517, 2.499999999999992006 ) ;
#11115=CIRCLE ( 'NONE', #9044, 6.999999999999999112 ) ;
#11125=ORIENTED_EDGE ( 'NONE', *, *, #7752, .F. ) ;
#11130=ORIENTED_EDGE ( 'NONE', *, *, #6317, .T. ) ;
#11142=DIRECTION ( 'NONE',  ( -1.000000000000000000, 6.162975822039154730E-33, 4.563833282352349791E-17 ) ) ;
#11164=AXIS2_PLACEMENT_3D ( 'NONE', #8508, #6528, #3631 ) ;
#11165=DIRECTION ( 'NONE',  ( -1.000000000000000000, 1.006188713385347367E-17, 3.844790828812615713E-17 ) ) ;
#11201=AXIS2_PLACEMENT_3D ( 'NONE', #1957, #7051, #2089 ) ;
#11227=VECTOR ( 'NONE', #11165, 1000.000000000000000 ) ;
#11230=CARTESIAN_POINT ( 'NONE',  ( 33.00000000000001421, 81.84122341717352356, -27.68198508464163510 ) ) ;
#11251=EDGE_CURVE ( 'NONE', #1961, #4493, #4275, .T. ) ;
#11252=CARTESIAN_POINT ( 'NONE',  ( 33.00000000000000711, 39.92642927056392210, -44.05727230799563898 ) ) ;
#11255=ORIENTED_EDGE ( 'NONE', *, *, #6317, .F. ) ;
#11260=AXIS2_PLACEMENT_3D ( 'NONE', #11674, #11805, #8825 ) ;
#11330=EDGE_LOOP ( 'NONE', ( #10197, #9993, #8364, #9054 ) ) ;
#11331=CARTESIAN_POINT ( 'NONE',  ( 33.00000000000001421, 39.34792583643766761, -24.06347054209567915 ) ) ;
#11348=DIRECTION ( 'NONE',  ( 0.000000000000000000, 0.000000000000000000, -1.000000000000000000 ) ) ;
#11354=ADVANCED_FACE ( 'NONE', ( #12213 ), #3517, .T. ) ;
#11356=CIRCLE ( 'NONE', #2738, 6.999999999999999112 ) ;
#11366=CARTESIAN_POINT ( 'NONE',  ( 33.00000000000001421, 81.84122341717352356, -27.68198508464163510 ) ) ;
#11376=CARTESIAN_POINT ( 'NONE',  ( 33.00000000000000711, 39.92642927056392210, -44.05727230799563898 ) ) ;
#11392=CARTESIAN_POINT ( 'NONE',  ( 27.00000000000001421, 81.84122341717352356, -12.68198508464164931 ) ) ;
#11426=FACE_OUTER_BOUND ( 'NONE', #3211, .T. ) ;
#11502=FACE_OUTER_BOUND ( 'NONE', #1215, .T. ) ;
#11505=DIRECTION ( 'NONE',  ( 0.000000000000000000, 0.000000000000000000, 1.000000000000000000 ) ) ;
#11517=AXIS2_PLACEMENT_3D ( 'NONE', #581, #1679, #11348 ) ;
#11525=DIRECTION ( 'NONE',  ( -1.000000000000000000, 1.006188713385347367E-17, 3.844790828812615713E-17 ) ) ;
#11554=DIRECTION ( 'NONE',  ( 0.000000000000000000, 0.000000000000000000, -1.000000000000000000 ) ) ;
#11555=CARTESIAN_POINT ( 'NONE',  ( 33.00000000000001421, 81.84122341717352356, -52.68198508464162444 ) ) ;
#11567=CARTESIAN_POINT ( 'NONE',  ( 27.00000000000001066, 39.92642927056392210, -44.05727230799563898 ) ) ;
#11573=VECTOR ( 'NONE', #4263, 1000.000000000000000 ) ;
#11668=SURFACE_STYLE_FILL_AREA ( #8705 ) ;
#11674=CARTESIAN_POINT ( 'NONE',  ( 27.00000000000001776, 48.04086878529346194, 39.26975893117280947 ) ) ;
#11676=EDGE_CURVE ( 'NONE', #9287, #12081, #11356, .T. ) ;
#11733=SHAPE_REPRESENTATION_RELATIONSHIP ( 'NONE' , 'NONE' ,  #2726, #1739 ) ;
#11749=EDGE_LOOP ( 'NONE', ( #9883, #1372, #6614, #5534 ) ) ;
#11767=EDGE_CURVE ( 'NONE', #2160, #10485, #7423, .T. ) ;
#11794=ORIENTED_EDGE ( 'NONE', *, *, #7391, .T. ) ;
#11805=DIRECTION ( 'NONE',  ( -1.000000000000000000, 6.162975822039154730E-33, 4.563833282352349791E-17 ) ) ;
#11837=ORIENTED_EDGE ( 'NONE', *, *, #12439, .T. ) ;
#11847=CARTESIAN_POINT ( 'NONE',  ( 33.00000000000001421, 39.34792583643766761, -17.06347054209568270 ) ) ;
#11899=LINE ( 'NONE', #423, #10837 ) ;
#11977=CARTESIAN_POINT ( 'NONE',  ( 33.00000000000000711, 39.92642927056392210, -44.05727230799563898 ) ) ;
#11989=FACE_OUTER_BOUND ( 'NONE', #2050, .T. ) ;
#11993=FACE_OUTER_BOUND ( 'NONE', #11749, .T. ) ;
#12027=AXIS2_PLACEMENT_3D ( 'NONE', #6692, #7889, #3851 ) ;
#12038=ADVANCED_FACE ( 'NONE', ( #11989 ), #3050, .T. ) ;
#12081=VERTEX_POINT ( 'NONE', #6 ) ;
#12101=ORIENTED_EDGE ( 'NONE', *, *, #9824, .F. ) ;
#12162=DIRECTION ( 'NONE',  ( -1.000000000000000000, 1.006188713385347367E-17, 3.844790828812615713E-17 ) ) ;
#12194=CARTESIAN_POINT ( 'NONE',  ( 27.00000000000001421, 39.34792583643766761, -14.56347054209569158 ) ) ;
#12197=AXIS2_PLACEMENT_3D ( 'NONE', #2198, #2929, #9835 ) ;
#12201=ORIENTED_EDGE ( 'NONE', *, *, #6754, .F. ) ;
#12213=FACE_OUTER_BOUND ( 'NONE', #223, .T. ) ;
#12276=ORIENTED_EDGE ( 'NONE', *, *, #6449, .T. ) ;
#12379=COLOUR_RGB ( '', 0.08235294, 0.09019608, 0.10196078) ;
#12393=ORIENTED_EDGE ( 'NONE', *, *, #2669, .T. ) ;
#12414=CYLINDRICAL_SURFACE ( 'NONE', #1336, 6.999999999999999112 ) ;
#12422=AXIS2_PLACEMENT_3D ( 'NONE', #5707, #7392, #6428 ) ;
#12439=EDGE_CURVE ( 'NONE', #7265, #9407, #1082, .T. ) ;
#12484=EDGE_CURVE ( 'NONE', #12081, #1191, #4381, .T. ) ;
#12542=EDGE_LOOP ( 'NONE', ( #11009, #11255 ) ) ;
#12550=ORIENTED_EDGE ( 'NONE', *, *, #3969, .T. ) ;
#12606=FACE_OUTER_BOUND ( 'NONE', #7345, .T. ) ;
#12621=CARTESIAN_POINT ( 'NONE',  ( 33.00000000000001421, 81.84122341717352356, -12.68198508464164931 ) ) ;
#12646=CARTESIAN_POINT ( 'NONE',  ( 27.00000000000001421, 81.84122341717352356, -42.68198508464162444 ) ) ;
#12648=FACE_OUTER_BOUND ( 'NONE', #748, .T. ) ;
#12657=EDGE_CURVE ( 'NONE', #3780, #10485, #10739, .T. ) ;
#12668=EDGE_CURVE ( 'NONE', #10794, #3780, #2380, .T. ) ;
#12706=SURFACE_SIDE_STYLE ('',( #11668 ) ) ;
ENDSEC;
END-ISO-10303-21;
